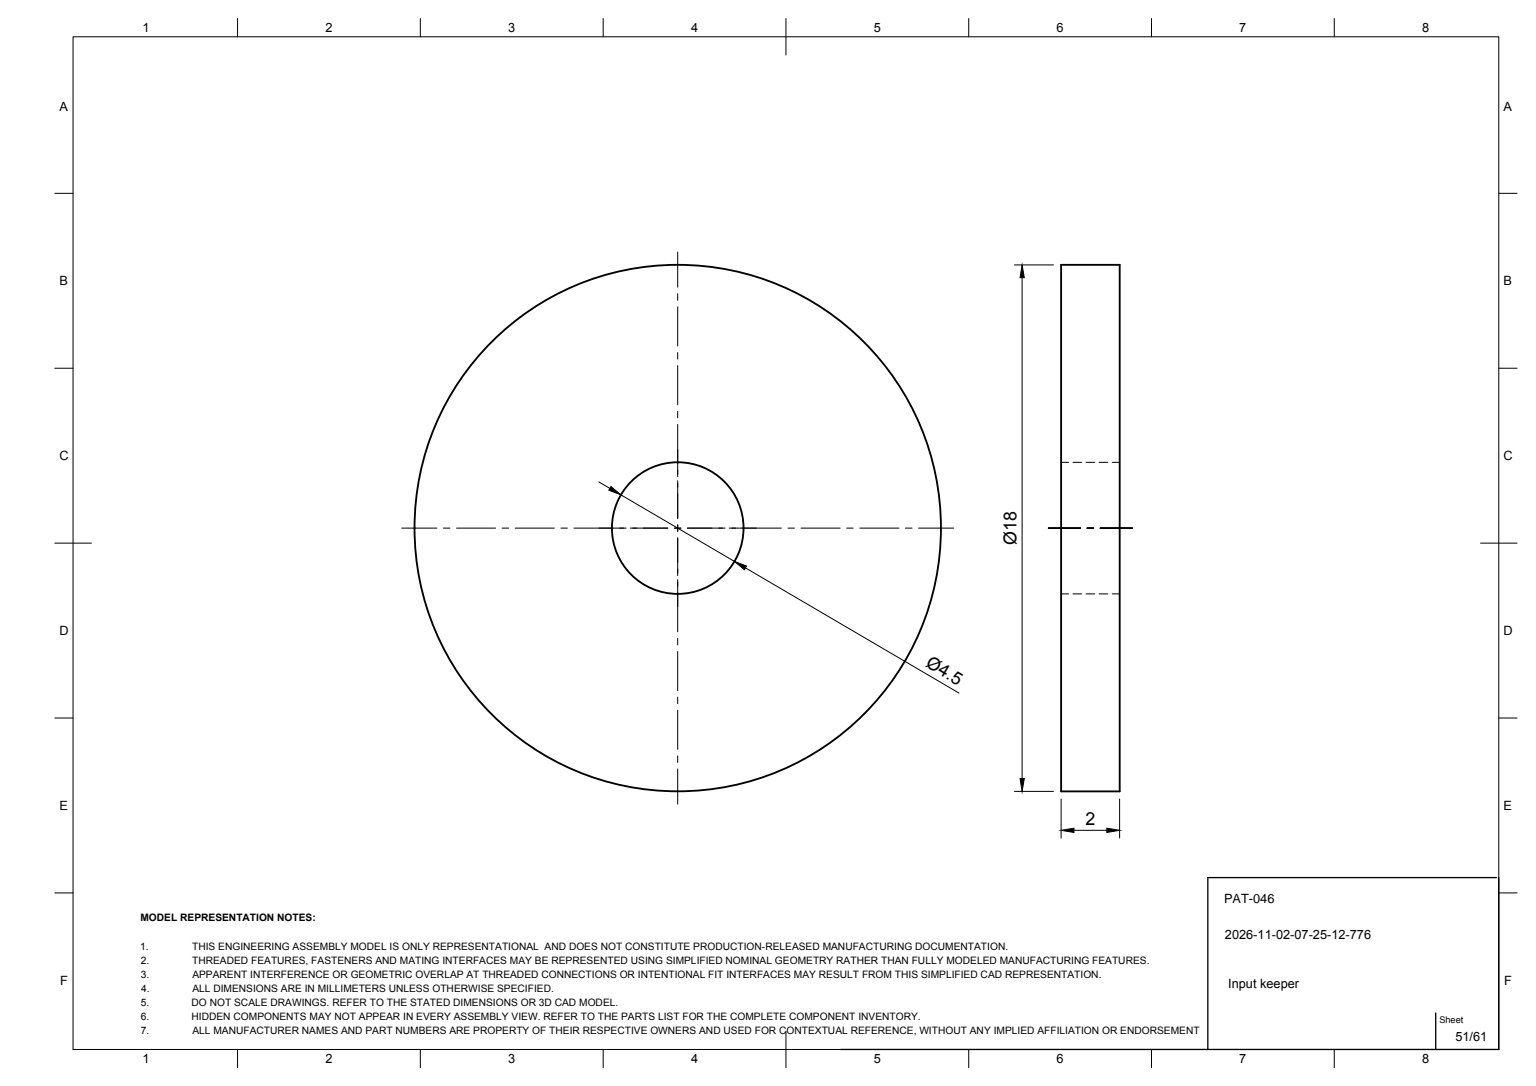
ISO-10303-21;
HEADER;
/* Generated by software containing ST-Developer
 * from STEP Tools, Inc. (www.steptools.com) 
 */

FILE_DESCRIPTION(
/* description */ ('Gear mesh backlash fixture'),
/* implementation_level */ '2;1');

FILE_NAME(
/* name */ 'Input keeper.step',
/* time_stamp */ '2026-10-28T03:26:00-07:00',
/* author */ (''),
/* organization */ (''),
/* preprocessor_version */ 'ST-DEVELOPER v20.2',
/* originating_system */ 'Autodesk Translation Framework v15.17.0.0',
/* authorisation */ '');

FILE_SCHEMA (('AUTOMOTIVE_DESIGN { 1 0 10303 214 3 1 1 }'));
ENDSEC;

DATA;
#10=MECHANICAL_DESIGN_GEOMETRIC_PRESENTATION_REPRESENTATION('',(#1070),#57900);
#955=SHAPE_REPRESENTATION_RELATIONSHIP('SRR','None',#58155,#1005);
#1005=ADVANCED_BREP_SHAPE_REPRESENTATION('',(#1133),#57888);
#1070=STYLED_ITEM('',(#58479),#1133);
#1133=MANIFOLD_SOLID_BREP('Body1',#13632);
#1306=FACE_BOUND('',#3066,.T.);
#1307=FACE_BOUND('',#3068,.T.);
#1576=PLANE('',#15126);
#1577=PLANE('',#15127);
#2135=FACE_OUTER_BOUND('',#3063,.T.);
#2136=FACE_OUTER_BOUND('',#3064,.T.);
#2137=FACE_OUTER_BOUND('',#3065,.T.);
#2138=FACE_OUTER_BOUND('',#3067,.T.);
#3063=EDGE_LOOP('',(#10837,#10838,#10839,#10840));
#3064=EDGE_LOOP('',(#10841,#10842,#10843,#10844));
#3065=EDGE_LOOP('',(#10845));
#3066=EDGE_LOOP('',(#10846));
#3067=EDGE_LOOP('',(#10847));
#3068=EDGE_LOOP('',(#10848));
#3918=LINE('',#22213,#4807);
#3919=LINE('',#22219,#4808);
#4807=VECTOR('',#17939,0.225);
#4808=VECTOR('',#17946,0.9);
#5613=CIRCLE('',#15121,0.225);
#5614=CIRCLE('',#15122,0.225);
#5615=CIRCLE('',#15124,0.9);
#5616=CIRCLE('',#15125,0.9);
#6444=VERTEX_POINT('',#22210);
#6445=VERTEX_POINT('',#22212);
#6446=VERTEX_POINT('',#22216);
#6447=VERTEX_POINT('',#22218);
#8005=EDGE_CURVE('',#6444,#6444,#5613,.T.);
#8006=EDGE_CURVE('',#6444,#6445,#3918,.T.);
#8007=EDGE_CURVE('',#6445,#6445,#5614,.T.);
#8008=EDGE_CURVE('',#6446,#6446,#5615,.T.);
#8009=EDGE_CURVE('',#6446,#6447,#3919,.T.);
#8010=EDGE_CURVE('',#6447,#6447,#5616,.T.);
#10837=ORIENTED_EDGE('',*,*,#8005,.F.);
#10838=ORIENTED_EDGE('',*,*,#8006,.T.);
#10839=ORIENTED_EDGE('',*,*,#8007,.T.);
#10840=ORIENTED_EDGE('',*,*,#8006,.F.);
#10841=ORIENTED_EDGE('',*,*,#8008,.F.);
#10842=ORIENTED_EDGE('',*,*,#8009,.T.);
#10843=ORIENTED_EDGE('',*,*,#8010,.T.);
#10844=ORIENTED_EDGE('',*,*,#8009,.F.);
#10845=ORIENTED_EDGE('',*,*,#8008,.T.);
#10846=ORIENTED_EDGE('',*,*,#8005,.T.);
#10847=ORIENTED_EDGE('',*,*,#8010,.F.);
#10848=ORIENTED_EDGE('',*,*,#8007,.F.);
#12729=CYLINDRICAL_SURFACE('',#15120,0.225);
#12730=CYLINDRICAL_SURFACE('',#15123,0.9);
#13252=ADVANCED_FACE('',(#2135),#12729,.F.);
#13253=ADVANCED_FACE('',(#2136),#12730,.T.);
#13254=ADVANCED_FACE('',(#2137,#1306),#1576,.T.);
#13255=ADVANCED_FACE('',(#2138,#1307),#1577,.F.);
#13632=CLOSED_SHELL('',(#13252,#13253,#13254,#13255));
#15119=AXIS2_PLACEMENT_3D('',#22208,#17933,#17934);
#15120=AXIS2_PLACEMENT_3D('',#22209,#17935,#17936);
#15121=AXIS2_PLACEMENT_3D('',#22211,#17937,#17938);
#15122=AXIS2_PLACEMENT_3D('',#22214,#17940,#17941);
#15123=AXIS2_PLACEMENT_3D('',#22215,#17942,#17943);
#15124=AXIS2_PLACEMENT_3D('',#22217,#17944,#17945);
#15125=AXIS2_PLACEMENT_3D('',#22220,#17947,#17948);
#15126=AXIS2_PLACEMENT_3D('',#22221,#17949,#17950);
#15127=AXIS2_PLACEMENT_3D('',#22222,#17951,#17952);
#17933=DIRECTION('axis',(0.,0.,1.));
#17934=DIRECTION('refdir',(1.,0.,0.));
#17935=DIRECTION('center_axis',(0.,0.,1.));
#17936=DIRECTION('ref_axis',(1.,0.,0.));
#17937=DIRECTION('center_axis',(0.,0.,-1.));
#17938=DIRECTION('ref_axis',(1.,0.,0.));
#17939=DIRECTION('',(0.,0.,-1.));
#17940=DIRECTION('center_axis',(0.,0.,-1.));
#17941=DIRECTION('ref_axis',(1.,0.,0.));
#17942=DIRECTION('center_axis',(0.,0.,1.));
#17943=DIRECTION('ref_axis',(1.,0.,0.));
#17944=DIRECTION('center_axis',(0.,0.,1.));
#17945=DIRECTION('ref_axis',(1.,0.,0.));
#17946=DIRECTION('',(0.,0.,-1.));
#17947=DIRECTION('center_axis',(0.,0.,1.));
#17948=DIRECTION('ref_axis',(1.,0.,0.));
#17949=DIRECTION('center_axis',(0.,0.,1.));
#17950=DIRECTION('ref_axis',(1.,0.,0.));
#17951=DIRECTION('center_axis',(0.,0.,1.));
#17952=DIRECTION('ref_axis',(1.,0.,0.));
#22208=CARTESIAN_POINT('',(0.,0.,0.));
#22209=CARTESIAN_POINT('Origin',(0.,0.,15.));
#22210=CARTESIAN_POINT('',(-0.225,-2.75545529808154E-17,15.2));
#22211=CARTESIAN_POINT('Origin',(0.,0.,15.2));
#22212=CARTESIAN_POINT('',(-0.225,-2.75545529808154E-17,15.));
#22213=CARTESIAN_POINT('',(-0.225,-2.75545529808154E-17,15.));
#22214=CARTESIAN_POINT('Origin',(0.,0.,15.));
#22215=CARTESIAN_POINT('Origin',(0.,0.,15.));
#22216=CARTESIAN_POINT('',(-0.9,-1.10218211923262E-16,15.2));
#22217=CARTESIAN_POINT('Origin',(0.,0.,15.2));
#22218=CARTESIAN_POINT('',(-0.9,-1.10218211923262E-16,15.));
#22219=CARTESIAN_POINT('',(-0.9,-1.10218211923262E-16,15.));
#22220=CARTESIAN_POINT('Origin',(0.,0.,15.));
#22221=CARTESIAN_POINT('Origin',(0.,0.,15.2));
#22222=CARTESIAN_POINT('Origin',(0.,0.,15.));
#57829=UNCERTAINTY_MEASURE_WITH_UNIT(LENGTH_MEASURE(0.001),#57901,
'DISTANCE_ACCURACY_VALUE',
'Maximum model space distance between geometric entities at asserted c
onnectivities');
#57841=UNCERTAINTY_MEASURE_WITH_UNIT(LENGTH_MEASURE(0.001),#57901,
'DISTANCE_ACCURACY_VALUE',
'Maximum model space distance between geometric entities at asserted c
onnectivities');
#57888=(
GEOMETRIC_REPRESENTATION_CONTEXT(3)
GLOBAL_UNCERTAINTY_ASSIGNED_CONTEXT((#57829))
GLOBAL_UNIT_ASSIGNED_CONTEXT((#57901,#57903,#57904))
REPRESENTATION_CONTEXT('','3D')
);
#57900=(
GEOMETRIC_REPRESENTATION_CONTEXT(3)
GLOBAL_UNCERTAINTY_ASSIGNED_CONTEXT((#57841))
GLOBAL_UNIT_ASSIGNED_CONTEXT((#57901,#57903,#57904))
REPRESENTATION_CONTEXT('','3D')
);
#57901=(
LENGTH_UNIT()
NAMED_UNIT(*)
SI_UNIT(.CENTI.,.METRE.)
);
#57903=(
NAMED_UNIT(*)
PLANE_ANGLE_UNIT()
SI_UNIT($,.RADIAN.)
);
#57904=(
NAMED_UNIT(*)
SI_UNIT($,.STERADIAN.)
SOLID_ANGLE_UNIT()
);
#57951=SHAPE_DEFINITION_REPRESENTATION(#58022,#58155);
#58022=PRODUCT_DEFINITION_SHAPE('',$,#58214);
#58155=SHAPE_REPRESENTATION('',(#15119),#57888);
#58167=PRODUCT_DEFINITION_CONTEXT('part definition',#58343,'design');
#58214=PRODUCT_DEFINITION('Input keeper','Input keeper',#58272,#58167);
#58272=PRODUCT_DEFINITION_FORMATION('',$,#58391);
#58343=APPLICATION_CONTEXT(
'Core Data for Automotive Mechanical Design Process');
#58344=PRODUCT_CONTEXT('part definition',#58343,'mechanical');
#58391=PRODUCT('Input keeper','Input keeper','Input keeper',(#58344));
#58473=COLOUR_RGB('Off White',0.89,0.88,0.83);
#58474=FILL_AREA_STYLE_COLOUR('',#58473);
#58475=FILL_AREA_STYLE('',(#58474));
#58476=SURFACE_STYLE_FILL_AREA(#58475);
#58477=SURFACE_SIDE_STYLE('',(#58476));
#58478=SURFACE_STYLE_USAGE(.BOTH.,#58477);
#58479=PRESENTATION_STYLE_ASSIGNMENT((#58478));
ENDSEC;
END-ISO-10303-21;
